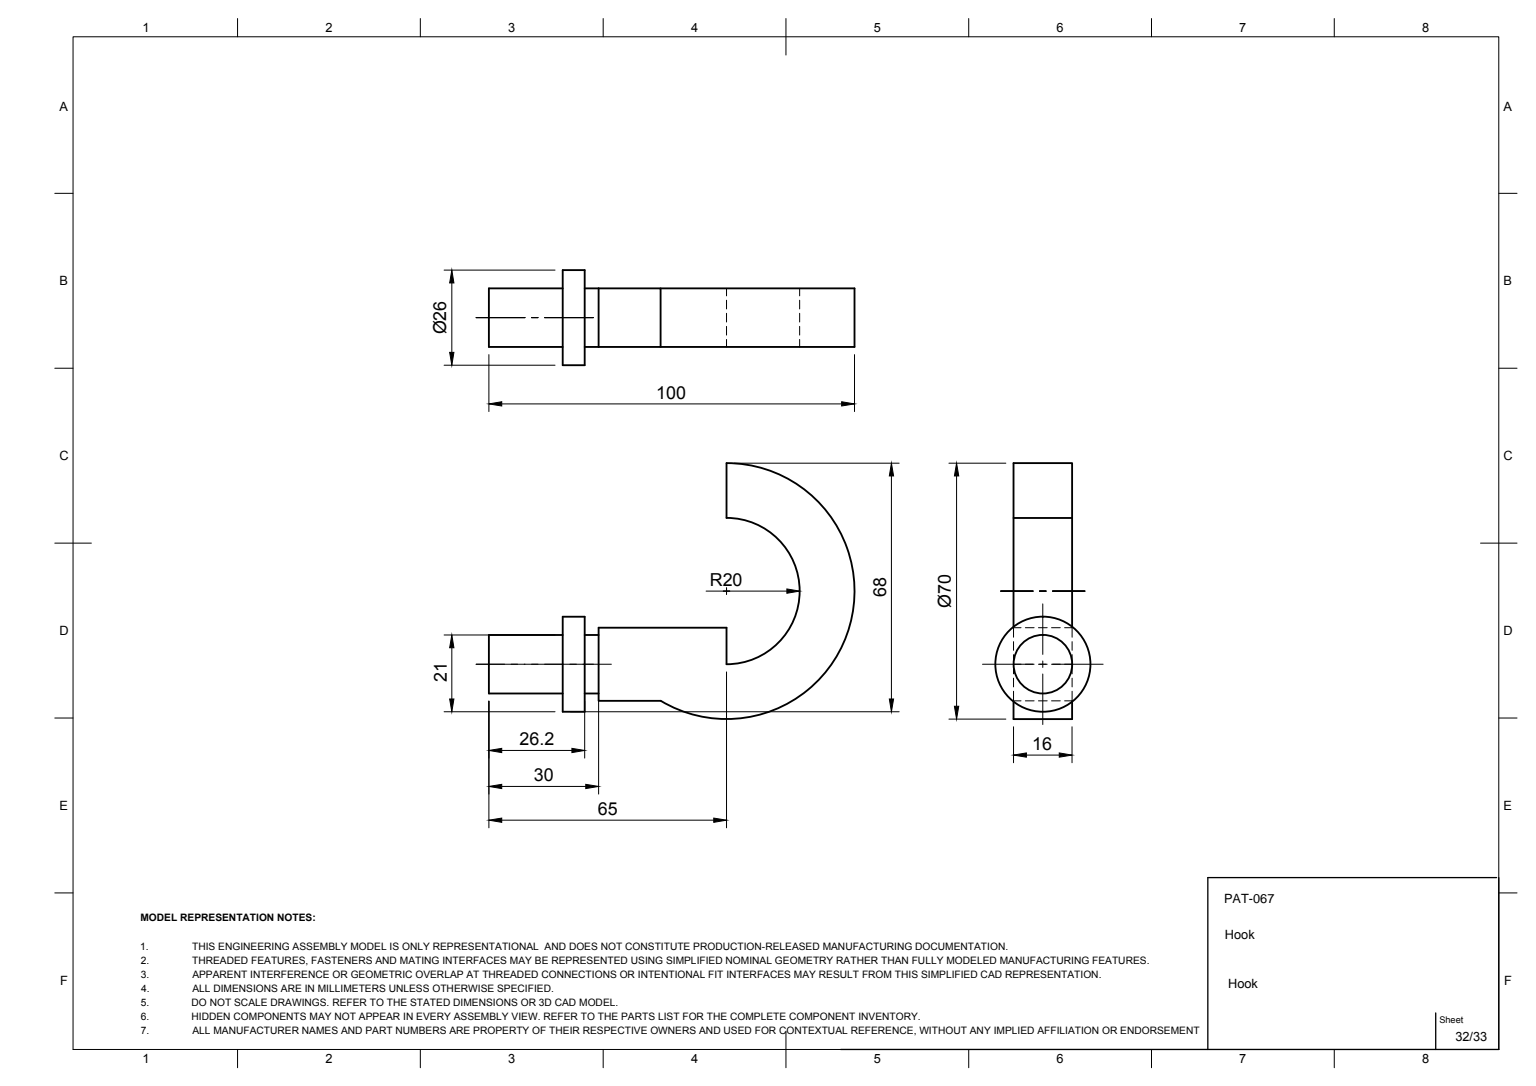
ISO-10303-21;
HEADER;
/* Generated by software containing ST-Developer
 * from STEP Tools, Inc. (www.steptools.com) 
 */

FILE_DESCRIPTION(
/* description */ ('Lifting hook block with sheave'),
/* implementation_level */ '2;1');

FILE_NAME(
/* name */ 'Hook.step',
/* time_stamp */ '2026-10-28T03:23:54-07:00',
/* author */ (''),
/* organization */ (''),
/* preprocessor_version */ 'ST-DEVELOPER v20.2',
/* originating_system */ 'Autodesk Translation Framework v15.17.0.0',
/* authorisation */ '');

FILE_SCHEMA (('AUTOMOTIVE_DESIGN { 1 0 10303 214 3 1 1 }'));
ENDSEC;

DATA;
#10=MECHANICAL_DESIGN_GEOMETRIC_PRESENTATION_REPRESENTATION('',(#385),#9391);
#317=SHAPE_REPRESENTATION_RELATIONSHIP('SRR','None',#9551,#347);
#347=ADVANCED_BREP_SHAPE_REPRESENTATION('',(#420),#9386);
#385=STYLED_ITEM('',(#9745),#420);
#420=MANIFOLD_SOLID_BREP('Body1',#4924);
#665=LINE('',#9161,#953);
#666=LINE('',#9164,#954);
#667=LINE('',#9173,#955);
#668=LINE('',#9177,#956);
#669=LINE('',#9179,#957);
#670=LINE('',#9180,#958);
#671=LINE('',#9183,#959);
#672=LINE('',#9185,#960);
#673=LINE('',#9186,#961);
#674=LINE('',#9190,#962);
#675=LINE('',#9191,#963);
#676=LINE('',#9192,#964);
#677=LINE('',#9196,#965);
#678=LINE('',#9198,#966);
#679=LINE('',#9200,#967);
#680=LINE('',#9201,#968);
#681=LINE('',#9203,#969);
#682=LINE('',#9207,#970);
#683=LINE('',#9212,#971);
#684=LINE('',#9214,#972);
#685=LINE('',#9217,#973);
#686=LINE('',#9220,#974);
#953=VECTOR('',#7378,1.3);
#954=VECTOR('',#7381,0.8);
#955=VECTOR('',#7392,0.8);
#956=VECTOR('',#7397,1.);
#957=VECTOR('',#7398,1.);
#958=VECTOR('',#7399,1.);
#959=VECTOR('',#7402,1.);
#960=VECTOR('',#7403,1.);
#961=VECTOR('',#7404,1.);
#962=VECTOR('',#7407,1.);
#963=VECTOR('',#7408,1.);
#964=VECTOR('',#7409,1.);
#965=VECTOR('',#7412,1.);
#966=VECTOR('',#7413,1.);
#967=VECTOR('',#7414,1.);
#968=VECTOR('',#7415,1.);
#969=VECTOR('',#7418,1.);
#970=VECTOR('',#7421,1.);
#971=VECTOR('',#7428,1.);
#972=VECTOR('',#7431,1.);
#973=VECTOR('',#7434,1.);
#974=VECTOR('',#7439,1.);
#1095=CYLINDRICAL_SURFACE('',#5862,1.3);
#1096=CYLINDRICAL_SURFACE('',#5863,0.8);
#1097=CYLINDRICAL_SURFACE('',#5867,0.8);
#1098=CYLINDRICAL_SURFACE('',#5877,2.);
#1099=CYLINDRICAL_SURFACE('',#5883,3.5);
#1212=FACE_BOUND('',#1871,.T.);
#1213=FACE_BOUND('',#1873,.T.);
#1476=FACE_OUTER_BOUND('',#1870,.T.);
#1477=FACE_OUTER_BOUND('',#1872,.T.);
#1478=FACE_OUTER_BOUND('',#1874,.T.);
#1479=FACE_OUTER_BOUND('',#1875,.T.);
#1480=FACE_OUTER_BOUND('',#1876,.T.);
#1481=FACE_OUTER_BOUND('',#1877,.T.);
#1482=FACE_OUTER_BOUND('',#1878,.T.);
#1483=FACE_OUTER_BOUND('',#1879,.T.);
#1484=FACE_OUTER_BOUND('',#1880,.T.);
#1485=FACE_OUTER_BOUND('',#1881,.T.);
#1486=FACE_OUTER_BOUND('',#1882,.T.);
#1487=FACE_OUTER_BOUND('',#1883,.T.);
#1488=FACE_OUTER_BOUND('',#1884,.T.);
#1489=FACE_OUTER_BOUND('',#1885,.T.);
#1490=FACE_OUTER_BOUND('',#1886,.T.);
#1491=FACE_OUTER_BOUND('',#1887,.T.);
#1870=EDGE_LOOP('',(#4306));
#1871=EDGE_LOOP('',(#4307));
#1872=EDGE_LOOP('',(#4308));
#1873=EDGE_LOOP('',(#4309));
#1874=EDGE_LOOP('',(#4310,#4311,#4312,#4313));
#1875=EDGE_LOOP('',(#4314,#4315,#4316,#4317,#4318,#4319));
#1876=EDGE_LOOP('',(#4320,#4321,#4322,#4323));
#1877=EDGE_LOOP('',(#4324));
#1878=EDGE_LOOP('',(#4325,#4326,#4327,#4328));
#1879=EDGE_LOOP('',(#4329,#4330,#4331,#4332,#4333));
#1880=EDGE_LOOP('',(#4334,#4335,#4336,#4337));
#1881=EDGE_LOOP('',(#4338,#4339,#4340,#4341));
#1882=EDGE_LOOP('',(#4342,#4343,#4344,#4345,#4346,#4347,#4348,#4349));
#1883=EDGE_LOOP('',(#4350,#4351,#4352,#4353));
#1884=EDGE_LOOP('',(#4354,#4355,#4356,#4357,#4358,#4359,#4360,#4361));
#1885=EDGE_LOOP('',(#4362,#4363,#4364,#4365));
#1886=EDGE_LOOP('',(#4366,#4367,#4368,#4369));
#1887=EDGE_LOOP('',(#4370,#4371,#4372,#4373));
#2182=CIRCLE('',#5857,1.3);
#2183=CIRCLE('',#5858,0.8);
#2184=CIRCLE('',#5860,1.3);
#2185=CIRCLE('',#5861,0.8);
#2186=CIRCLE('',#5864,0.8);
#2187=CIRCLE('',#5865,0.8);
#2188=CIRCLE('',#5866,0.8);
#2189=CIRCLE('',#5868,0.8);
#2190=CIRCLE('',#5875,2.);
#2191=CIRCLE('',#5876,3.5);
#2192=CIRCLE('',#5878,2.);
#2193=CIRCLE('',#5880,3.5);
#2571=VERTEX_POINT('',#9151);
#2572=VERTEX_POINT('',#9153);
#2573=VERTEX_POINT('',#9156);
#2574=VERTEX_POINT('',#9158);
#2575=VERTEX_POINT('',#9163);
#2576=VERTEX_POINT('',#9165);
#2577=VERTEX_POINT('',#9167);
#2578=VERTEX_POINT('',#9171);
#2579=VERTEX_POINT('',#9176);
#2580=VERTEX_POINT('',#9178);
#2581=VERTEX_POINT('',#9182);
#2582=VERTEX_POINT('',#9184);
#2583=VERTEX_POINT('',#9188);
#2584=VERTEX_POINT('',#9189);
#2585=VERTEX_POINT('',#9194);
#2586=VERTEX_POINT('',#9195);
#2587=VERTEX_POINT('',#9197);
#2588=VERTEX_POINT('',#9199);
#2589=VERTEX_POINT('',#9204);
#2590=VERTEX_POINT('',#9206);
#2591=VERTEX_POINT('',#9210);
#2592=VERTEX_POINT('',#9215);
#3157=EDGE_CURVE('',#2571,#2571,#2182,.T.);
#3158=EDGE_CURVE('',#2572,#2572,#2183,.T.);
#3159=EDGE_CURVE('',#2573,#2573,#2184,.T.);
#3160=EDGE_CURVE('',#2574,#2574,#2185,.T.);
#3161=EDGE_CURVE('',#2571,#2573,#665,.T.);
#3162=EDGE_CURVE('',#2574,#2575,#666,.T.);
#3163=EDGE_CURVE('',#2576,#2575,#2186,.T.);
#3164=EDGE_CURVE('',#2577,#2576,#2187,.T.);
#3165=EDGE_CURVE('',#2575,#2577,#2188,.T.);
#3166=EDGE_CURVE('',#2578,#2578,#2189,.T.);
#3167=EDGE_CURVE('',#2578,#2572,#667,.T.);
#3168=EDGE_CURVE('',#2579,#2576,#668,.T.);
#3169=EDGE_CURVE('',#2579,#2580,#669,.T.);
#3170=EDGE_CURVE('',#2577,#2580,#670,.T.);
#3171=EDGE_CURVE('',#2581,#2577,#671,.T.);
#3172=EDGE_CURVE('',#2582,#2581,#672,.T.);
#3173=EDGE_CURVE('',#2576,#2582,#673,.T.);
#3174=EDGE_CURVE('',#2583,#2584,#674,.T.);
#3175=EDGE_CURVE('',#2582,#2583,#675,.T.);
#3176=EDGE_CURVE('',#2584,#2581,#676,.T.);
#3177=EDGE_CURVE('',#2585,#2586,#677,.T.);
#3178=EDGE_CURVE('',#2587,#2585,#678,.T.);
#3179=EDGE_CURVE('',#2588,#2587,#679,.T.);
#3180=EDGE_CURVE('',#2586,#2588,#680,.T.);
#3181=EDGE_CURVE('',#2580,#2587,#681,.T.);
#3182=EDGE_CURVE('',#2585,#2589,#2190,.T.);
#3183=EDGE_CURVE('',#2589,#2590,#682,.T.);
#3184=EDGE_CURVE('',#2590,#2584,#2191,.T.);
#3185=EDGE_CURVE('',#2586,#2591,#2192,.T.);
#3186=EDGE_CURVE('',#2591,#2589,#683,.T.);
#3187=EDGE_CURVE('',#2588,#2579,#684,.T.);
#3188=EDGE_CURVE('',#2592,#2583,#2193,.T.);
#3189=EDGE_CURVE('',#2592,#2591,#685,.T.);
#3190=EDGE_CURVE('',#2590,#2592,#686,.T.);
#4306=ORIENTED_EDGE('',*,*,#3157,.T.);
#4307=ORIENTED_EDGE('',*,*,#3158,.F.);
#4308=ORIENTED_EDGE('',*,*,#3159,.F.);
#4309=ORIENTED_EDGE('',*,*,#3160,.F.);
#4310=ORIENTED_EDGE('',*,*,#3157,.F.);
#4311=ORIENTED_EDGE('',*,*,#3161,.T.);
#4312=ORIENTED_EDGE('',*,*,#3159,.T.);
#4313=ORIENTED_EDGE('',*,*,#3161,.F.);
#4314=ORIENTED_EDGE('',*,*,#3160,.T.);
#4315=ORIENTED_EDGE('',*,*,#3162,.T.);
#4316=ORIENTED_EDGE('',*,*,#3163,.F.);
#4317=ORIENTED_EDGE('',*,*,#3164,.F.);
#4318=ORIENTED_EDGE('',*,*,#3165,.F.);
#4319=ORIENTED_EDGE('',*,*,#3162,.F.);
#4320=ORIENTED_EDGE('',*,*,#3166,.F.);
#4321=ORIENTED_EDGE('',*,*,#3167,.T.);
#4322=ORIENTED_EDGE('',*,*,#3158,.T.);
#4323=ORIENTED_EDGE('',*,*,#3167,.F.);
#4324=ORIENTED_EDGE('',*,*,#3166,.T.);
#4325=ORIENTED_EDGE('',*,*,#3164,.T.);
#4326=ORIENTED_EDGE('',*,*,#3168,.F.);
#4327=ORIENTED_EDGE('',*,*,#3169,.T.);
#4328=ORIENTED_EDGE('',*,*,#3170,.F.);
#4329=ORIENTED_EDGE('',*,*,#3163,.T.);
#4330=ORIENTED_EDGE('',*,*,#3165,.T.);
#4331=ORIENTED_EDGE('',*,*,#3171,.F.);
#4332=ORIENTED_EDGE('',*,*,#3172,.F.);
#4333=ORIENTED_EDGE('',*,*,#3173,.F.);
#4334=ORIENTED_EDGE('',*,*,#3174,.F.);
#4335=ORIENTED_EDGE('',*,*,#3175,.F.);
#4336=ORIENTED_EDGE('',*,*,#3172,.T.);
#4337=ORIENTED_EDGE('',*,*,#3176,.F.);
#4338=ORIENTED_EDGE('',*,*,#3177,.F.);
#4339=ORIENTED_EDGE('',*,*,#3178,.F.);
#4340=ORIENTED_EDGE('',*,*,#3179,.F.);
#4341=ORIENTED_EDGE('',*,*,#3180,.F.);
#4342=ORIENTED_EDGE('',*,*,#3181,.T.);
#4343=ORIENTED_EDGE('',*,*,#3178,.T.);
#4344=ORIENTED_EDGE('',*,*,#3182,.T.);
#4345=ORIENTED_EDGE('',*,*,#3183,.T.);
#4346=ORIENTED_EDGE('',*,*,#3184,.T.);
#4347=ORIENTED_EDGE('',*,*,#3176,.T.);
#4348=ORIENTED_EDGE('',*,*,#3171,.T.);
#4349=ORIENTED_EDGE('',*,*,#3170,.T.);
#4350=ORIENTED_EDGE('',*,*,#3177,.T.);
#4351=ORIENTED_EDGE('',*,*,#3185,.T.);
#4352=ORIENTED_EDGE('',*,*,#3186,.T.);
#4353=ORIENTED_EDGE('',*,*,#3182,.F.);
#4354=ORIENTED_EDGE('',*,*,#3187,.T.);
#4355=ORIENTED_EDGE('',*,*,#3168,.T.);
#4356=ORIENTED_EDGE('',*,*,#3173,.T.);
#4357=ORIENTED_EDGE('',*,*,#3175,.T.);
#4358=ORIENTED_EDGE('',*,*,#3188,.F.);
#4359=ORIENTED_EDGE('',*,*,#3189,.T.);
#4360=ORIENTED_EDGE('',*,*,#3185,.F.);
#4361=ORIENTED_EDGE('',*,*,#3180,.T.);
#4362=ORIENTED_EDGE('',*,*,#3187,.F.);
#4363=ORIENTED_EDGE('',*,*,#3179,.T.);
#4364=ORIENTED_EDGE('',*,*,#3181,.F.);
#4365=ORIENTED_EDGE('',*,*,#3169,.F.);
#4366=ORIENTED_EDGE('',*,*,#3190,.F.);
#4367=ORIENTED_EDGE('',*,*,#3183,.F.);
#4368=ORIENTED_EDGE('',*,*,#3186,.F.);
#4369=ORIENTED_EDGE('',*,*,#3189,.F.);
#4370=ORIENTED_EDGE('',*,*,#3174,.T.);
#4371=ORIENTED_EDGE('',*,*,#3184,.F.);
#4372=ORIENTED_EDGE('',*,*,#3190,.T.);
#4373=ORIENTED_EDGE('',*,*,#3188,.T.);
#4575=PLANE('',#5856);
#4576=PLANE('',#5859);
#4577=PLANE('',#5869);
#4578=PLANE('',#5870);
#4579=PLANE('',#5871);
#4580=PLANE('',#5872);
#4581=PLANE('',#5873);
#4582=PLANE('',#5874);
#4583=PLANE('',#5879);
#4584=PLANE('',#5881);
#4585=PLANE('',#5882);
#4852=ADVANCED_FACE('',(#1476,#1212),#4575,.T.);
#4853=ADVANCED_FACE('',(#1477,#1213),#4576,.F.);
#4854=ADVANCED_FACE('',(#1478),#1095,.T.);
#4855=ADVANCED_FACE('',(#1479),#1096,.T.);
#4856=ADVANCED_FACE('',(#1480),#1097,.T.);
#4857=ADVANCED_FACE('',(#1481),#4577,.T.);
#4858=ADVANCED_FACE('',(#1482),#4578,.T.);
#4859=ADVANCED_FACE('',(#1483),#4579,.T.);
#4860=ADVANCED_FACE('',(#1484),#4580,.T.);
#4861=ADVANCED_FACE('',(#1485),#4581,.T.);
#4862=ADVANCED_FACE('',(#1486),#4582,.T.);
#4863=ADVANCED_FACE('',(#1487),#1098,.F.);
#4864=ADVANCED_FACE('',(#1488),#4583,.F.);
#4865=ADVANCED_FACE('',(#1489),#4584,.F.);
#4866=ADVANCED_FACE('',(#1490),#4585,.F.);
#4867=ADVANCED_FACE('',(#1491),#1099,.T.);
#4924=CLOSED_SHELL('',(#4852,#4853,#4854,#4855,#4856,#4857,#4858,#4859,
#4860,#4861,#4862,#4863,#4864,#4865,#4866,#4867));
#5855=AXIS2_PLACEMENT_3D('',#9149,#7362,#7363);
#5856=AXIS2_PLACEMENT_3D('',#9150,#7364,#7365);
#5857=AXIS2_PLACEMENT_3D('',#9152,#7366,#7367);
#5858=AXIS2_PLACEMENT_3D('',#9154,#7368,#7369);
#5859=AXIS2_PLACEMENT_3D('',#9155,#7370,#7371);
#5860=AXIS2_PLACEMENT_3D('',#9157,#7372,#7373);
#5861=AXIS2_PLACEMENT_3D('',#9159,#7374,#7375);
#5862=AXIS2_PLACEMENT_3D('',#9160,#7376,#7377);
#5863=AXIS2_PLACEMENT_3D('',#9162,#7379,#7380);
#5864=AXIS2_PLACEMENT_3D('',#9166,#7382,#7383);
#5865=AXIS2_PLACEMENT_3D('',#9168,#7384,#7385);
#5866=AXIS2_PLACEMENT_3D('',#9169,#7386,#7387);
#5867=AXIS2_PLACEMENT_3D('',#9170,#7388,#7389);
#5868=AXIS2_PLACEMENT_3D('',#9172,#7390,#7391);
#5869=AXIS2_PLACEMENT_3D('',#9174,#7393,#7394);
#5870=AXIS2_PLACEMENT_3D('',#9175,#7395,#7396);
#5871=AXIS2_PLACEMENT_3D('',#9181,#7400,#7401);
#5872=AXIS2_PLACEMENT_3D('',#9187,#7405,#7406);
#5873=AXIS2_PLACEMENT_3D('',#9193,#7410,#7411);
#5874=AXIS2_PLACEMENT_3D('',#9202,#7416,#7417);
#5875=AXIS2_PLACEMENT_3D('',#9205,#7419,#7420);
#5876=AXIS2_PLACEMENT_3D('',#9208,#7422,#7423);
#5877=AXIS2_PLACEMENT_3D('',#9209,#7424,#7425);
#5878=AXIS2_PLACEMENT_3D('',#9211,#7426,#7427);
#5879=AXIS2_PLACEMENT_3D('',#9213,#7429,#7430);
#5880=AXIS2_PLACEMENT_3D('',#9216,#7432,#7433);
#5881=AXIS2_PLACEMENT_3D('',#9218,#7435,#7436);
#5882=AXIS2_PLACEMENT_3D('',#9219,#7437,#7438);
#5883=AXIS2_PLACEMENT_3D('',#9221,#7440,#7441);
#7362=DIRECTION('axis',(0.,0.,1.));
#7363=DIRECTION('refdir',(1.,0.,0.));
#7364=DIRECTION('center_axis',(0.,0.,1.));
#7365=DIRECTION('ref_axis',(1.,0.,0.));
#7366=DIRECTION('center_axis',(0.,0.,1.));
#7367=DIRECTION('ref_axis',(1.,0.,0.));
#7368=DIRECTION('center_axis',(0.,0.,1.));
#7369=DIRECTION('ref_axis',(1.,0.,0.));
#7370=DIRECTION('center_axis',(0.,0.,1.));
#7371=DIRECTION('ref_axis',(1.,0.,0.));
#7372=DIRECTION('center_axis',(0.,0.,1.));
#7373=DIRECTION('ref_axis',(1.,0.,0.));
#7374=DIRECTION('center_axis',(0.,0.,-1.));
#7375=DIRECTION('ref_axis',(1.,0.,0.));
#7376=DIRECTION('center_axis',(0.,0.,1.));
#7377=DIRECTION('ref_axis',(1.,0.,0.));
#7378=DIRECTION('',(0.,0.,-1.));
#7379=DIRECTION('center_axis',(0.,0.,1.));
#7380=DIRECTION('ref_axis',(1.,0.,0.));
#7381=DIRECTION('',(0.,0.,-1.));
#7382=DIRECTION('center_axis',(0.,0.,-1.));
#7383=DIRECTION('ref_axis',(1.,0.,0.));
#7384=DIRECTION('center_axis',(0.,0.,-1.));
#7385=DIRECTION('ref_axis',(1.,0.,0.));
#7386=DIRECTION('center_axis',(0.,0.,-1.));
#7387=DIRECTION('ref_axis',(1.,0.,0.));
#7388=DIRECTION('center_axis',(0.,0.,1.));
#7389=DIRECTION('ref_axis',(1.,0.,0.));
#7390=DIRECTION('center_axis',(0.,0.,1.));
#7391=DIRECTION('ref_axis',(1.,0.,0.));
#7392=DIRECTION('',(0.,0.,-1.));
#7393=DIRECTION('center_axis',(0.,0.,1.));
#7394=DIRECTION('ref_axis',(1.,0.,0.));
#7395=DIRECTION('center_axis',(0.,0.,1.));
#7396=DIRECTION('ref_axis',(1.,0.,0.));
#7397=DIRECTION('',(-1.,0.,0.));
#7398=DIRECTION('',(0.,1.,0.));
#7399=DIRECTION('',(1.,0.,0.));
#7400=DIRECTION('center_axis',(0.,0.,1.));
#7401=DIRECTION('ref_axis',(1.,0.,0.));
#7402=DIRECTION('',(1.,0.,0.));
#7403=DIRECTION('',(0.,1.,0.));
#7404=DIRECTION('',(-1.,0.,0.));
#7405=DIRECTION('center_axis',(-1.,0.,0.));
#7406=DIRECTION('ref_axis',(0.,0.,1.));
#7407=DIRECTION('',(0.,1.,0.));
#7408=DIRECTION('',(0.,0.,-1.));
#7409=DIRECTION('',(0.,0.,1.));
#7410=DIRECTION('center_axis',(0.,0.,-1.));
#7411=DIRECTION('ref_axis',(-1.,0.,0.));
#7412=DIRECTION('',(0.,-1.,0.));
#7413=DIRECTION('',(-1.,0.,0.));
#7414=DIRECTION('',(0.,1.,0.));
#7415=DIRECTION('',(1.,0.,0.));
#7416=DIRECTION('center_axis',(0.,1.,0.));
#7417=DIRECTION('ref_axis',(1.,0.,0.));
#7418=DIRECTION('',(0.,0.,-1.));
#7419=DIRECTION('center_axis',(0.,-1.,0.));
#7420=DIRECTION('ref_axis',(1.,0.,0.));
#7421=DIRECTION('',(1.,0.,0.));
#7422=DIRECTION('center_axis',(0.,1.,0.));
#7423=DIRECTION('ref_axis',(1.,0.,0.));
#7424=DIRECTION('center_axis',(0.,1.,0.));
#7425=DIRECTION('ref_axis',(1.,0.,0.));
#7426=DIRECTION('center_axis',(0.,-1.,0.));
#7427=DIRECTION('ref_axis',(1.,0.,0.));
#7428=DIRECTION('',(0.,1.,0.));
#7429=DIRECTION('center_axis',(0.,1.,0.));
#7430=DIRECTION('ref_axis',(1.,0.,0.));
#7431=DIRECTION('',(0.,0.,1.));
#7432=DIRECTION('center_axis',(0.,1.,0.));
#7433=DIRECTION('ref_axis',(1.,0.,0.));
#7434=DIRECTION('',(-1.,0.,0.));
#7435=DIRECTION('center_axis',(-1.,0.,0.));
#7436=DIRECTION('ref_axis',(0.,0.,1.));
#7437=DIRECTION('center_axis',(0.,0.,-1.));
#7438=DIRECTION('ref_axis',(-1.,0.,0.));
#7439=DIRECTION('',(0.,-1.,0.));
#7440=DIRECTION('center_axis',(0.,1.,0.));
#7441=DIRECTION('ref_axis',(-0.267261241912424,0.,-0.963624111659432));
#9149=CARTESIAN_POINT('',(0.,0.,0.));
#9150=CARTESIAN_POINT('Origin',(0.,0.,4.48));
#9151=CARTESIAN_POINT('',(-1.3,-1.59204083889156E-16,4.48));
#9152=CARTESIAN_POINT('Origin',(0.,0.,4.48));
#9153=CARTESIAN_POINT('',(-0.8,-9.79717439317883E-17,4.48));
#9154=CARTESIAN_POINT('Origin',(0.,0.,4.48));
#9155=CARTESIAN_POINT('Origin',(0.,0.,3.88));
#9156=CARTESIAN_POINT('',(-1.3,-1.59204083889156E-16,3.88));
#9157=CARTESIAN_POINT('Origin',(0.,0.,3.88));
#9158=CARTESIAN_POINT('',(-0.8,9.79717439317883E-17,3.88));
#9159=CARTESIAN_POINT('Origin',(0.,0.,3.88));
#9160=CARTESIAN_POINT('Origin',(0.,0.,3.88));
#9161=CARTESIAN_POINT('',(-1.3,-1.59204083889156E-16,3.88));
#9162=CARTESIAN_POINT('Origin',(0.,0.,3.));
#9163=CARTESIAN_POINT('',(-0.8,-9.79717439317883E-17,3.5));
#9164=CARTESIAN_POINT('',(-0.8,-9.79717439317883E-17,3.));
#9165=CARTESIAN_POINT('',(0.,-0.8,3.5));
#9166=CARTESIAN_POINT('Origin',(0.,0.,3.5));
#9167=CARTESIAN_POINT('',(0.,0.8,3.5));
#9168=CARTESIAN_POINT('Origin',(0.,0.,3.5));
#9169=CARTESIAN_POINT('Origin',(0.,0.,3.5));
#9170=CARTESIAN_POINT('Origin',(0.,0.,3.));
#9171=CARTESIAN_POINT('',(-0.8,-9.79717439317883E-17,6.5));
#9172=CARTESIAN_POINT('Origin',(0.,0.,6.5));
#9173=CARTESIAN_POINT('',(-0.8,-9.79717439317883E-17,3.));
#9174=CARTESIAN_POINT('Origin',(0.,0.,6.5));
#9175=CARTESIAN_POINT('Origin',(-1.,-0.8,3.5));
#9176=CARTESIAN_POINT('',(1.,-0.8,3.5));
#9177=CARTESIAN_POINT('',(1.,-0.8,3.5));
#9178=CARTESIAN_POINT('',(1.,0.8,3.5));
#9179=CARTESIAN_POINT('',(1.,-0.8,3.5));
#9180=CARTESIAN_POINT('',(1.,0.8,3.5));
#9181=CARTESIAN_POINT('Origin',(-1.,-0.8,3.5));
#9182=CARTESIAN_POINT('',(-1.,0.8,3.5));
#9183=CARTESIAN_POINT('',(1.,0.8,3.5));
#9184=CARTESIAN_POINT('',(-1.,-0.8,3.5));
#9185=CARTESIAN_POINT('',(-1.,-0.8,3.5));
#9186=CARTESIAN_POINT('',(1.,-0.8,3.5));
#9187=CARTESIAN_POINT('Origin',(-1.,-0.8,0.));
#9188=CARTESIAN_POINT('',(-1.,-0.8,1.80277563773199));
#9189=CARTESIAN_POINT('',(-1.,0.8,1.80277563773199));
#9190=CARTESIAN_POINT('',(-1.,-0.8,1.80277563773199));
#9191=CARTESIAN_POINT('',(-1.,-0.8,3.5));
#9192=CARTESIAN_POINT('',(-1.,0.8,3.5));
#9193=CARTESIAN_POINT('Origin',(1.,-0.8,0.));
#9194=CARTESIAN_POINT('',(0.,0.8,0.));
#9195=CARTESIAN_POINT('',(0.,-0.8,0.));
#9196=CARTESIAN_POINT('',(0.,-0.8,0.));
#9197=CARTESIAN_POINT('',(1.,0.8,0.));
#9198=CARTESIAN_POINT('',(-1.,0.8,0.));
#9199=CARTESIAN_POINT('',(1.,-0.8,0.));
#9200=CARTESIAN_POINT('',(1.,-0.8,0.));
#9201=CARTESIAN_POINT('',(-1.,-0.8,0.));
#9202=CARTESIAN_POINT('Origin',(2.,0.8,0.));
#9203=CARTESIAN_POINT('',(1.,0.8,0.));
#9204=CARTESIAN_POINT('',(4.,0.8,0.));
#9205=CARTESIAN_POINT('Origin',(2.,0.8,0.));
#9206=CARTESIAN_POINT('',(5.5,0.8,0.));
#9207=CARTESIAN_POINT('',(4.,0.8,0.));
#9208=CARTESIAN_POINT('Origin',(2.,0.8,0.));
#9209=CARTESIAN_POINT('Origin',(2.,-0.8,0.));
#9210=CARTESIAN_POINT('',(4.,-0.8,0.));
#9211=CARTESIAN_POINT('Origin',(2.,-0.8,0.));
#9212=CARTESIAN_POINT('',(4.,-0.8,0.));
#9213=CARTESIAN_POINT('Origin',(2.,-0.8,0.));
#9214=CARTESIAN_POINT('',(1.,-0.8,0.));
#9215=CARTESIAN_POINT('',(5.5,-0.8,0.));
#9216=CARTESIAN_POINT('Origin',(2.,-0.8,0.));
#9217=CARTESIAN_POINT('',(4.,-0.8,0.));
#9218=CARTESIAN_POINT('Origin',(1.,-0.9,0.));
#9219=CARTESIAN_POINT('Origin',(6.,-0.9,0.));
#9220=CARTESIAN_POINT('',(5.5,-0.8,0.));
#9221=CARTESIAN_POINT('Origin',(2.,-0.8,0.));
#9349=UNCERTAINTY_MEASURE_WITH_UNIT(LENGTH_MEASURE(0.001),#9392,
'DISTANCE_ACCURACY_VALUE',
'Maximum model space distance between geometric entities at asserted c
onnectivities');
#9354=UNCERTAINTY_MEASURE_WITH_UNIT(LENGTH_MEASURE(0.001),#9392,
'DISTANCE_ACCURACY_VALUE',
'Maximum model space distance between geometric entities at asserted c
onnectivities');
#9386=(
GEOMETRIC_REPRESENTATION_CONTEXT(3)
GLOBAL_UNCERTAINTY_ASSIGNED_CONTEXT((#9349))
GLOBAL_UNIT_ASSIGNED_CONTEXT((#9392,#9394,#9395))
REPRESENTATION_CONTEXT('','3D')
);
#9391=(
GEOMETRIC_REPRESENTATION_CONTEXT(3)
GLOBAL_UNCERTAINTY_ASSIGNED_CONTEXT((#9354))
GLOBAL_UNIT_ASSIGNED_CONTEXT((#9392,#9394,#9395))
REPRESENTATION_CONTEXT('','3D')
);
#9392=(
LENGTH_UNIT()
NAMED_UNIT(*)
SI_UNIT(.CENTI.,.METRE.)
);
#9394=(
NAMED_UNIT(*)
PLANE_ANGLE_UNIT()
SI_UNIT($,.RADIAN.)
);
#9395=(
NAMED_UNIT(*)
SI_UNIT($,.STERADIAN.)
SOLID_ANGLE_UNIT()
);
#9427=SHAPE_DEFINITION_REPRESENTATION(#9507,#9551);
#9507=PRODUCT_DEFINITION_SHAPE('',$,#9588);
#9551=SHAPE_REPRESENTATION('',(#5855),#9386);
#9556=PRODUCT_DEFINITION_CONTEXT('part definition',#9666,'design');
#9588=PRODUCT_DEFINITION('Hook','Hook',#9624,#9556);
#9624=PRODUCT_DEFINITION_FORMATION('',$,#9699);
#9666=APPLICATION_CONTEXT(
'Core Data for Automotive Mechanical Design Process');
#9667=PRODUCT_CONTEXT('part definition',#9666,'mechanical');
#9699=PRODUCT('Hook','Hook','Hook',(#9667));
#9739=COLOUR_RGB('Light Blue',0.38,0.62,0.78);
#9740=FILL_AREA_STYLE_COLOUR('',#9739);
#9741=FILL_AREA_STYLE('',(#9740));
#9742=SURFACE_STYLE_FILL_AREA(#9741);
#9743=SURFACE_SIDE_STYLE('',(#9742));
#9744=SURFACE_STYLE_USAGE(.BOTH.,#9743);
#9745=PRESENTATION_STYLE_ASSIGNMENT((#9744));
ENDSEC;
END-ISO-10303-21;
